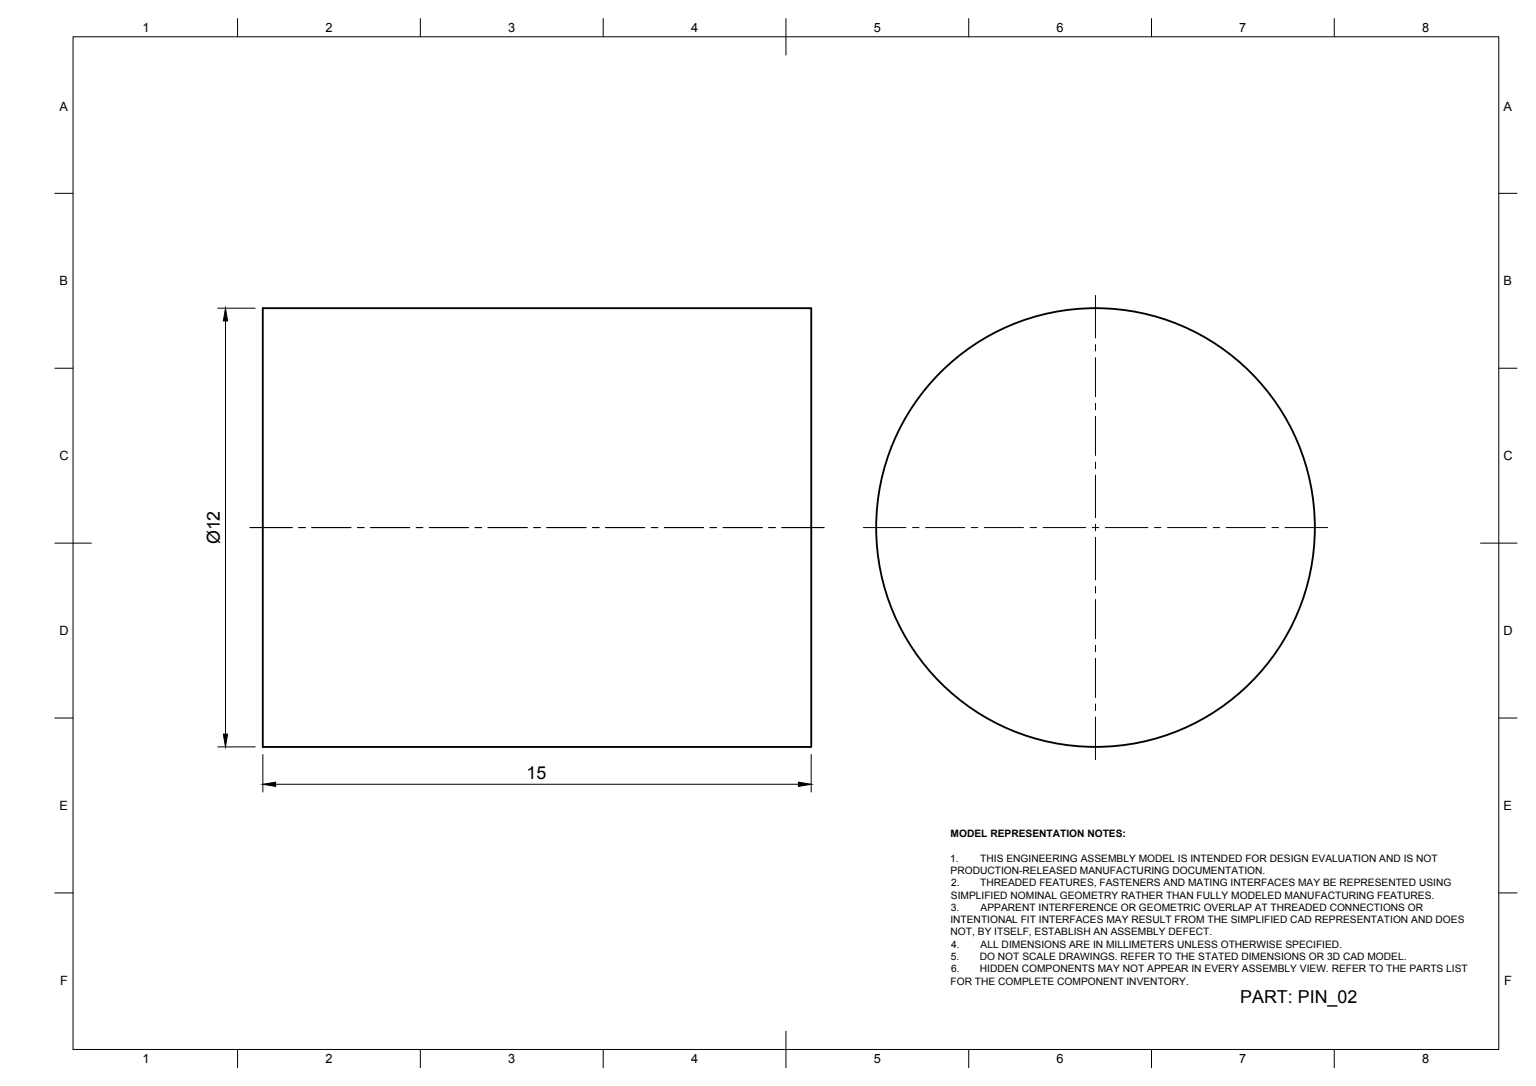
ISO-10303-21;
HEADER;
/* Generated by software containing ST-Developer
 * from STEP Tools, Inc. (www.steptools.com) 
 */

FILE_DESCRIPTION(
/* description */ (''),
/* implementation_level */ '2;1');

FILE_NAME(
/* name */ 'Pin_02.step',
/* time_stamp */ '2026-09-20T22:38:01+06:00',
/* author */ (''),
/* organization */ (''),
/* preprocessor_version */ 'ST-DEVELOPER v20.2',
/* originating_system */ 'Autodesk Translation Framework v15.15.0.0',
/* authorisation */ '');

FILE_SCHEMA (('AUTOMOTIVE_DESIGN { 1 0 10303 214 3 1 1 }'));
ENDSEC;

DATA;
#10=MECHANICAL_DESIGN_GEOMETRIC_PRESENTATION_REPRESENTATION('',(#88),#4079);
#72=SHAPE_REPRESENTATION_RELATIONSHIP('SRR','None',#4115,#80);
#80=ADVANCED_BREP_SHAPE_REPRESENTATION('',(#96),#4075);
#88=STYLED_ITEM('',(#4159),#96);
#96=MANIFOLD_SOLID_BREP('Pin_02',#1447);
#161=CIRCLE('',#1660,6.);
#162=CIRCLE('',#1661,6.);
#193=CYLINDRICAL_SURFACE('',#1659,6.);
#261=FACE_OUTER_BOUND('',#351,.T.);
#262=FACE_OUTER_BOUND('',#352,.T.);
#263=FACE_OUTER_BOUND('',#353,.T.);
#351=EDGE_LOOP('',(#1237,#1238,#1239,#1240));
#352=EDGE_LOOP('',(#1241));
#353=EDGE_LOOP('',(#1242));
#456=LINE('',#3973,#569);
#569=VECTOR('',#2025,6.);
#700=VERTEX_POINT('',#3970);
#701=VERTEX_POINT('',#3972);
#883=EDGE_CURVE('',#700,#700,#161,.T.);
#884=EDGE_CURVE('',#700,#701,#456,.T.);
#885=EDGE_CURVE('',#701,#701,#162,.T.);
#1237=ORIENTED_EDGE('',*,*,#883,.F.);
#1238=ORIENTED_EDGE('',*,*,#884,.T.);
#1239=ORIENTED_EDGE('',*,*,#885,.T.);
#1240=ORIENTED_EDGE('',*,*,#884,.F.);
#1241=ORIENTED_EDGE('',*,*,#883,.T.);
#1242=ORIENTED_EDGE('',*,*,#885,.F.);
#1343=PLANE('',#1662);
#1344=PLANE('',#1663);
#1423=ADVANCED_FACE('',(#261),#193,.T.);
#1424=ADVANCED_FACE('',(#262),#1343,.T.);
#1425=ADVANCED_FACE('',(#263),#1344,.F.);
#1447=CLOSED_SHELL('',(#1423,#1424,#1425));
#1658=AXIS2_PLACEMENT_3D('',#3968,#2019,#2020);
#1659=AXIS2_PLACEMENT_3D('',#3969,#2021,#2022);
#1660=AXIS2_PLACEMENT_3D('',#3971,#2023,#2024);
#1661=AXIS2_PLACEMENT_3D('',#3974,#2026,#2027);
#1662=AXIS2_PLACEMENT_3D('',#3975,#2028,#2029);
#1663=AXIS2_PLACEMENT_3D('',#3976,#2030,#2031);
#2019=DIRECTION('axis',(0.,0.,1.));
#2020=DIRECTION('refdir',(1.,0.,0.));
#2021=DIRECTION('center_axis',(0.,-1.,0.));
#2022=DIRECTION('ref_axis',(1.,0.,0.));
#2023=DIRECTION('center_axis',(0.,-1.,0.));
#2024=DIRECTION('ref_axis',(1.,0.,0.));
#2025=DIRECTION('',(0.,1.,0.));
#2026=DIRECTION('center_axis',(0.,-1.,0.));
#2027=DIRECTION('ref_axis',(1.,0.,0.));
#2028=DIRECTION('center_axis',(0.,-1.,0.));
#2029=DIRECTION('ref_axis',(1.,0.,0.));
#2030=DIRECTION('center_axis',(0.,-1.,0.));
#2031=DIRECTION('ref_axis',(1.,0.,0.));
#3968=CARTESIAN_POINT('',(0.,0.,0.));
#3969=CARTESIAN_POINT('Origin',(73.2288574389116,5.,87.4952777324745));
#3970=CARTESIAN_POINT('',(67.2288574389116,-10.,87.4952777324745));
#3971=CARTESIAN_POINT('Origin',(73.2288574389116,-10.,87.4952777324745));
#3972=CARTESIAN_POINT('',(67.2288574389116,5.,87.4952777324745));
#3973=CARTESIAN_POINT('',(67.2288574389116,5.,87.4952777324745));
#3974=CARTESIAN_POINT('Origin',(73.2288574389116,5.,87.4952777324745));
#3975=CARTESIAN_POINT('Origin',(73.2288574389116,-10.,87.4952777324745));
#3976=CARTESIAN_POINT('Origin',(73.2288574389116,5.,87.4952777324745));
#4065=UNCERTAINTY_MEASURE_WITH_UNIT(LENGTH_MEASURE(0.01),#4080,
'DISTANCE_ACCURACY_VALUE',
'Maximum model space distance between geometric entities at asserted c
onnectivities');
#4069=UNCERTAINTY_MEASURE_WITH_UNIT(LENGTH_MEASURE(0.01),#4080,
'DISTANCE_ACCURACY_VALUE',
'Maximum model space distance between geometric entities at asserted c
onnectivities');
#4075=(
GEOMETRIC_REPRESENTATION_CONTEXT(3)
GLOBAL_UNCERTAINTY_ASSIGNED_CONTEXT((#4065))
GLOBAL_UNIT_ASSIGNED_CONTEXT((#4080,#4082,#4083))
REPRESENTATION_CONTEXT('','3D')
);
#4079=(
GEOMETRIC_REPRESENTATION_CONTEXT(3)
GLOBAL_UNCERTAINTY_ASSIGNED_CONTEXT((#4069))
GLOBAL_UNIT_ASSIGNED_CONTEXT((#4080,#4082,#4083))
REPRESENTATION_CONTEXT('','3D')
);
#4080=(
LENGTH_UNIT()
NAMED_UNIT(*)
SI_UNIT(.MILLI.,.METRE.)
);
#4082=(
NAMED_UNIT(*)
PLANE_ANGLE_UNIT()
SI_UNIT($,.RADIAN.)
);
#4083=(
NAMED_UNIT(*)
SI_UNIT($,.STERADIAN.)
SOLID_ANGLE_UNIT()
);
#4089=SHAPE_DEFINITION_REPRESENTATION(#4098,#4115);
#4098=PRODUCT_DEFINITION_SHAPE('',$,#4125);
#4115=SHAPE_REPRESENTATION('',(#1658),#4075);
#4119=PRODUCT_DEFINITION_CONTEXT('part definition',#4148,'design');
#4125=PRODUCT_DEFINITION('Pin_02','Pin_02',#4134,#4119);
#4134=PRODUCT_DEFINITION_FORMATION('',$,#4155);
#4148=APPLICATION_CONTEXT(
'Core Data for Automotive Mechanical Design Process');
#4149=PRODUCT_CONTEXT('part definition',#4148,'mechanical');
#4155=PRODUCT('Pin_02','Pin_02',$,(#4149));
#4159=PRESENTATION_STYLE_ASSIGNMENT((#4163));
#4163=SURFACE_STYLE_USAGE(.BOTH.,#4167);
#4167=SURFACE_SIDE_STYLE('',(#4171));
#4171=SURFACE_STYLE_FILL_AREA(#4175);
#4175=FILL_AREA_STYLE('Steel - Satin',(#4179));
#4179=FILL_AREA_STYLE_COLOUR('Steel - Satin',#4183);
#4183=COLOUR_RGB('Steel - Satin', 0.40784314, 0.44705882, 0.49803922);
ENDSEC;
END-ISO-10303-21;
